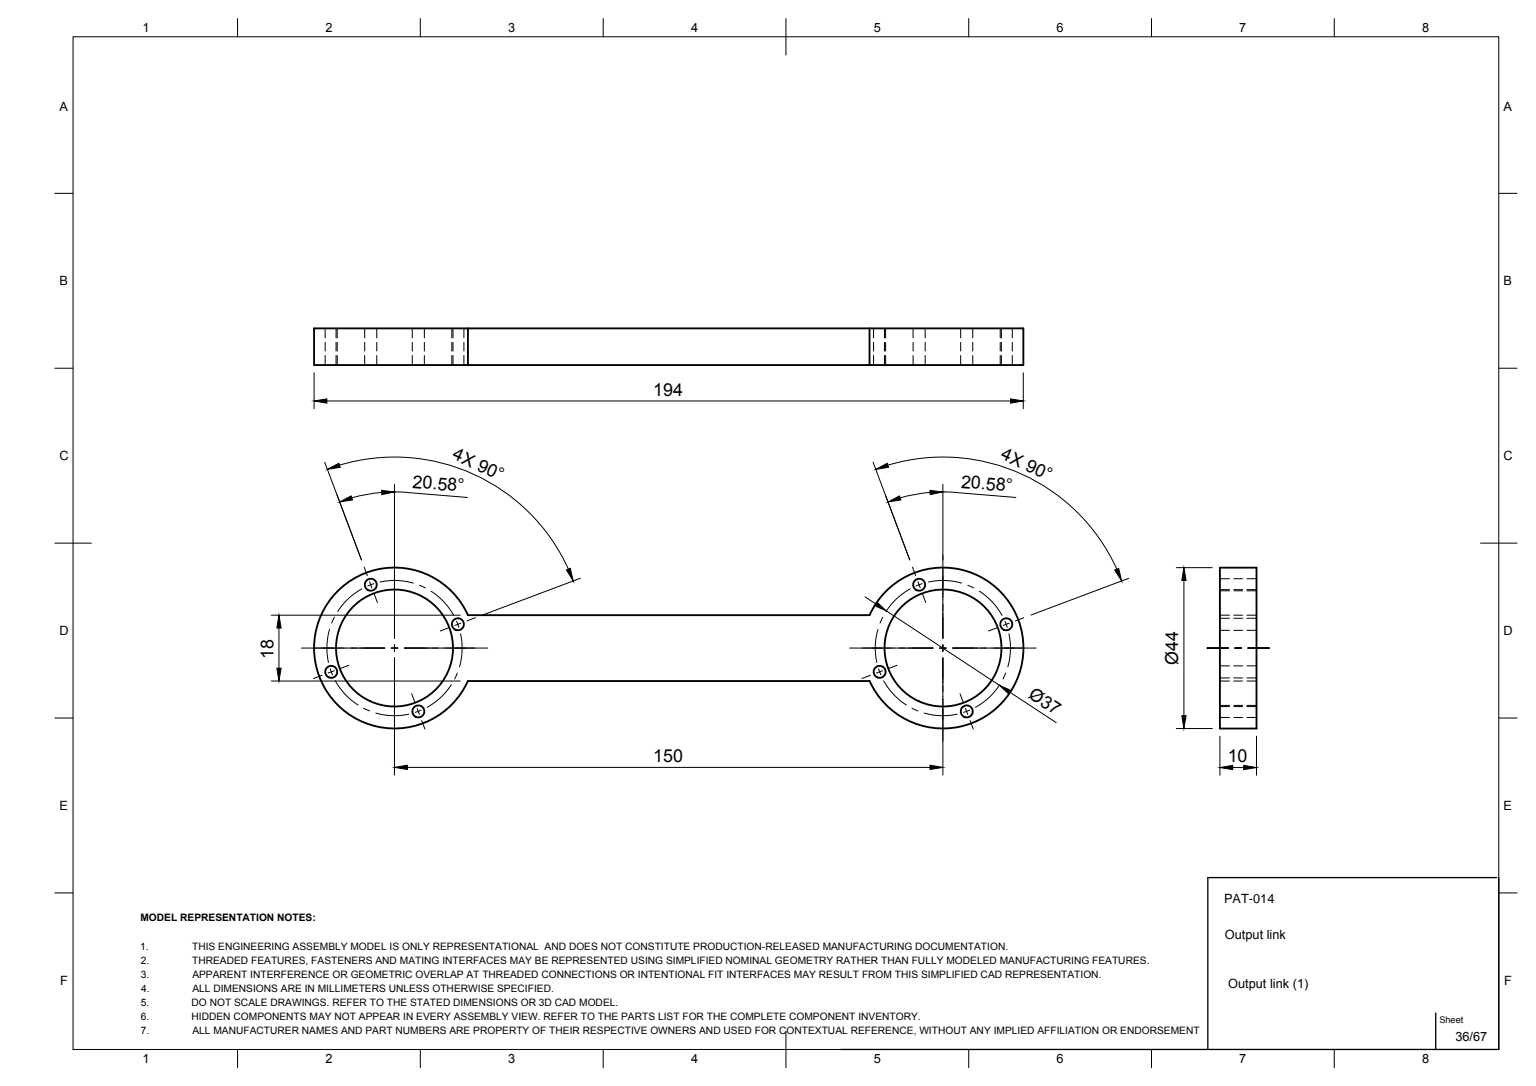
ISO-10303-21;
HEADER;
/* Generated by software containing ST-Developer
 * from STEP Tools, Inc. (www.steptools.com) 
 */

FILE_DESCRIPTION(
/* description */ ('Bin tilter linkage'),
/* implementation_level */ '2;1');

FILE_NAME(
/* name */ 'Output link (1).step',
/* time_stamp */ '2026-10-28T03:26:24-07:00',
/* author */ (''),
/* organization */ (''),
/* preprocessor_version */ 'ST-DEVELOPER v20.2',
/* originating_system */ 'Autodesk Translation Framework v15.17.0.0',
/* authorisation */ '');

FILE_SCHEMA (('AUTOMOTIVE_DESIGN { 1 0 10303 214 3 1 1 }'));
ENDSEC;

DATA;
#10=MECHANICAL_DESIGN_GEOMETRIC_PRESENTATION_REPRESENTATION('',(#913),#23728);
#701=SHAPE_REPRESENTATION_RELATIONSHIP('SRR','None',#24167,#807);
#807=ADVANCED_BREP_SHAPE_REPRESENTATION('',(#1026),#23667);
#913=STYLED_ITEM('',(#24779),#1026);
#1026=MANIFOLD_SOLID_BREP('Body1',#12444);
#1310=FACE_BOUND('',#3275,.T.);
#1311=FACE_BOUND('',#3276,.T.);
#1312=FACE_BOUND('',#3277,.T.);
#1313=FACE_BOUND('',#3278,.T.);
#1314=FACE_BOUND('',#3279,.T.);
#1315=FACE_BOUND('',#3280,.T.);
#1316=FACE_BOUND('',#3281,.T.);
#1317=FACE_BOUND('',#3282,.T.);
#1318=FACE_BOUND('',#3283,.T.);
#1319=FACE_BOUND('',#3284,.T.);
#1320=FACE_BOUND('',#3293,.T.);
#1321=FACE_BOUND('',#3294,.T.);
#1322=FACE_BOUND('',#3295,.T.);
#1323=FACE_BOUND('',#3296,.T.);
#1324=FACE_BOUND('',#3297,.T.);
#1325=FACE_BOUND('',#3298,.T.);
#1326=FACE_BOUND('',#3299,.T.);
#1327=FACE_BOUND('',#3300,.T.);
#1328=FACE_BOUND('',#3301,.T.);
#1329=FACE_BOUND('',#3302,.T.);
#1677=PLANE('',#14507);
#1678=PLANE('',#14508);
#1679=PLANE('',#14527);
#1680=PLANE('',#14528);
#2267=FACE_OUTER_BOUND('',#3267,.T.);
#2268=FACE_OUTER_BOUND('',#3268,.T.);
#2269=FACE_OUTER_BOUND('',#3269,.T.);
#2270=FACE_OUTER_BOUND('',#3270,.T.);
#2271=FACE_OUTER_BOUND('',#3271,.T.);
#2272=FACE_OUTER_BOUND('',#3272,.T.);
#2273=FACE_OUTER_BOUND('',#3273,.T.);
#2274=FACE_OUTER_BOUND('',#3274,.T.);
#2275=FACE_OUTER_BOUND('',#3285,.T.);
#2276=FACE_OUTER_BOUND('',#3286,.T.);
#2277=FACE_OUTER_BOUND('',#3287,.T.);
#2278=FACE_OUTER_BOUND('',#3288,.T.);
#2279=FACE_OUTER_BOUND('',#3289,.T.);
#2280=FACE_OUTER_BOUND('',#3290,.T.);
#2281=FACE_OUTER_BOUND('',#3291,.T.);
#2282=FACE_OUTER_BOUND('',#3292,.T.);
#3267=EDGE_LOOP('',(#9793,#9794,#9795,#9796));
#3268=EDGE_LOOP('',(#9797,#9798,#9799,#9800));
#3269=EDGE_LOOP('',(#9801,#9802,#9803,#9804));
#3270=EDGE_LOOP('',(#9805,#9806,#9807,#9808));
#3271=EDGE_LOOP('',(#9809,#9810,#9811,#9812));
#3272=EDGE_LOOP('',(#9813,#9814,#9815,#9816));
#3273=EDGE_LOOP('',(#9817,#9818,#9819,#9820));
#3274=EDGE_LOOP('',(#9821,#9822,#9823,#9824));
#3275=EDGE_LOOP('',(#9825));
#3276=EDGE_LOOP('',(#9826));
#3277=EDGE_LOOP('',(#9827));
#3278=EDGE_LOOP('',(#9828));
#3279=EDGE_LOOP('',(#9829));
#3280=EDGE_LOOP('',(#9830));
#3281=EDGE_LOOP('',(#9831));
#3282=EDGE_LOOP('',(#9832));
#3283=EDGE_LOOP('',(#9833));
#3284=EDGE_LOOP('',(#9834));
#3285=EDGE_LOOP('',(#9835,#9836,#9837,#9838));
#3286=EDGE_LOOP('',(#9839,#9840,#9841,#9842));
#3287=EDGE_LOOP('',(#9843,#9844,#9845,#9846));
#3288=EDGE_LOOP('',(#9847,#9848,#9849,#9850));
#3289=EDGE_LOOP('',(#9851,#9852,#9853,#9854));
#3290=EDGE_LOOP('',(#9855,#9856,#9857,#9858));
#3291=EDGE_LOOP('',(#9859,#9860,#9861,#9862));
#3292=EDGE_LOOP('',(#9863,#9864,#9865,#9866));
#3293=EDGE_LOOP('',(#9867));
#3294=EDGE_LOOP('',(#9868));
#3295=EDGE_LOOP('',(#9869));
#3296=EDGE_LOOP('',(#9870));
#3297=EDGE_LOOP('',(#9871));
#3298=EDGE_LOOP('',(#9872));
#3299=EDGE_LOOP('',(#9873));
#3300=EDGE_LOOP('',(#9874));
#3301=EDGE_LOOP('',(#9875));
#3302=EDGE_LOOP('',(#9876));
#4179=LINE('',#21364,#4854);
#4180=LINE('',#21370,#4855);
#4181=LINE('',#21376,#4856);
#4182=LINE('',#21382,#4857);
#4183=LINE('',#21388,#4858);
#4184=LINE('',#21393,#4859);
#4185=LINE('',#21397,#4860);
#4186=LINE('',#21401,#4861);
#4187=LINE('',#21403,#4862);
#4188=LINE('',#21404,#4863);
#4189=LINE('',#21407,#4864);
#4190=LINE('',#21422,#4865);
#4191=LINE('',#21426,#4866);
#4192=LINE('',#21430,#4867);
#4193=LINE('',#21434,#4868);
#4194=LINE('',#21438,#4869);
#4195=LINE('',#21441,#4870);
#4196=LINE('',#21444,#4871);
#4854=VECTOR('',#17434,0.164999999999999);
#4855=VECTOR('',#17441,0.164999999999999);
#4856=VECTOR('',#17448,0.164999999999999);
#4857=VECTOR('',#17455,0.164999999999999);
#4858=VECTOR('',#17462,1.6);
#4859=VECTOR('',#17467,1.);
#4860=VECTOR('',#17470,1.);
#4861=VECTOR('',#17475,1.);
#4862=VECTOR('',#17476,1.);
#4863=VECTOR('',#17477,1.);
#4864=VECTOR('',#17480,1.);
#4865=VECTOR('',#17497,0.164999999999999);
#4866=VECTOR('',#17502,0.164999999999999);
#4867=VECTOR('',#17507,0.164999999999999);
#4868=VECTOR('',#17512,0.164999999999999);
#4869=VECTOR('',#17517,1.6);
#4870=VECTOR('',#17520,1.);
#4871=VECTOR('',#17525,1.);
#5579=CIRCLE('',#14490,0.164999999999999);
#5580=CIRCLE('',#14491,0.164999999999999);
#5581=CIRCLE('',#14493,0.164999999999999);
#5582=CIRCLE('',#14494,0.164999999999999);
#5583=CIRCLE('',#14496,0.164999999999999);
#5584=CIRCLE('',#14497,0.164999999999999);
#5585=CIRCLE('',#14499,0.164999999999999);
#5586=CIRCLE('',#14500,0.164999999999999);
#5587=CIRCLE('',#14502,1.6);
#5588=CIRCLE('',#14503,1.6);
#5589=CIRCLE('',#14505,2.2);
#5590=CIRCLE('',#14506,2.2);
#5591=CIRCLE('',#14509,2.2);
#5592=CIRCLE('',#14510,1.6);
#5593=CIRCLE('',#14511,0.164999999999999);
#5594=CIRCLE('',#14512,0.164999999999999);
#5595=CIRCLE('',#14513,0.164999999999999);
#5596=CIRCLE('',#14514,0.164999999999999);
#5597=CIRCLE('',#14516,0.164999999999999);
#5598=CIRCLE('',#14518,0.164999999999999);
#5599=CIRCLE('',#14520,0.164999999999999);
#5600=CIRCLE('',#14522,0.164999999999999);
#5601=CIRCLE('',#14524,1.6);
#5602=CIRCLE('',#14526,2.2);
#6429=VERTEX_POINT('',#21361);
#6430=VERTEX_POINT('',#21363);
#6431=VERTEX_POINT('',#21367);
#6432=VERTEX_POINT('',#21369);
#6433=VERTEX_POINT('',#21373);
#6434=VERTEX_POINT('',#21375);
#6435=VERTEX_POINT('',#21379);
#6436=VERTEX_POINT('',#21381);
#6437=VERTEX_POINT('',#21385);
#6438=VERTEX_POINT('',#21387);
#6439=VERTEX_POINT('',#21391);
#6440=VERTEX_POINT('',#21392);
#6441=VERTEX_POINT('',#21394);
#6442=VERTEX_POINT('',#21396);
#6443=VERTEX_POINT('',#21400);
#6444=VERTEX_POINT('',#21402);
#6445=VERTEX_POINT('',#21406);
#6446=VERTEX_POINT('',#21409);
#6447=VERTEX_POINT('',#21411);
#6448=VERTEX_POINT('',#21413);
#6449=VERTEX_POINT('',#21415);
#6450=VERTEX_POINT('',#21417);
#6451=VERTEX_POINT('',#21420);
#6452=VERTEX_POINT('',#21424);
#6453=VERTEX_POINT('',#21428);
#6454=VERTEX_POINT('',#21432);
#6455=VERTEX_POINT('',#21436);
#6456=VERTEX_POINT('',#21440);
#7636=EDGE_CURVE('',#6429,#6429,#5579,.T.);
#7637=EDGE_CURVE('',#6429,#6430,#4179,.T.);
#7638=EDGE_CURVE('',#6430,#6430,#5580,.T.);
#7639=EDGE_CURVE('',#6431,#6431,#5581,.T.);
#7640=EDGE_CURVE('',#6431,#6432,#4180,.T.);
#7641=EDGE_CURVE('',#6432,#6432,#5582,.T.);
#7642=EDGE_CURVE('',#6433,#6433,#5583,.T.);
#7643=EDGE_CURVE('',#6433,#6434,#4181,.T.);
#7644=EDGE_CURVE('',#6434,#6434,#5584,.T.);
#7645=EDGE_CURVE('',#6435,#6435,#5585,.T.);
#7646=EDGE_CURVE('',#6435,#6436,#4182,.T.);
#7647=EDGE_CURVE('',#6436,#6436,#5586,.T.);
#7648=EDGE_CURVE('',#6437,#6437,#5587,.T.);
#7649=EDGE_CURVE('',#6437,#6438,#4183,.T.);
#7650=EDGE_CURVE('',#6438,#6438,#5588,.T.);
#7651=EDGE_CURVE('',#6439,#6440,#4184,.T.);
#7652=EDGE_CURVE('',#6439,#6441,#5589,.T.);
#7653=EDGE_CURVE('',#6442,#6441,#4185,.T.);
#7654=EDGE_CURVE('',#6440,#6442,#5590,.T.);
#7655=EDGE_CURVE('',#6443,#6440,#4186,.T.);
#7656=EDGE_CURVE('',#6443,#6444,#4187,.T.);
#7657=EDGE_CURVE('',#6444,#6439,#4188,.T.);
#7658=EDGE_CURVE('',#6442,#6445,#4189,.T.);
#7659=EDGE_CURVE('',#6445,#6443,#5591,.T.);
#7660=EDGE_CURVE('',#6446,#6446,#5592,.T.);
#7661=EDGE_CURVE('',#6447,#6447,#5593,.T.);
#7662=EDGE_CURVE('',#6448,#6448,#5594,.T.);
#7663=EDGE_CURVE('',#6449,#6449,#5595,.T.);
#7664=EDGE_CURVE('',#6450,#6450,#5596,.T.);
#7665=EDGE_CURVE('',#6451,#6451,#5597,.T.);
#7666=EDGE_CURVE('',#6451,#6450,#4190,.T.);
#7667=EDGE_CURVE('',#6452,#6452,#5598,.T.);
#7668=EDGE_CURVE('',#6452,#6449,#4191,.T.);
#7669=EDGE_CURVE('',#6453,#6453,#5599,.T.);
#7670=EDGE_CURVE('',#6453,#6448,#4192,.T.);
#7671=EDGE_CURVE('',#6454,#6454,#5600,.T.);
#7672=EDGE_CURVE('',#6454,#6447,#4193,.T.);
#7673=EDGE_CURVE('',#6455,#6455,#5601,.T.);
#7674=EDGE_CURVE('',#6455,#6446,#4194,.T.);
#7675=EDGE_CURVE('',#6456,#6445,#4195,.T.);
#7676=EDGE_CURVE('',#6456,#6444,#5602,.T.);
#7677=EDGE_CURVE('',#6441,#6456,#4196,.T.);
#9793=ORIENTED_EDGE('',*,*,#7636,.F.);
#9794=ORIENTED_EDGE('',*,*,#7637,.T.);
#9795=ORIENTED_EDGE('',*,*,#7638,.F.);
#9796=ORIENTED_EDGE('',*,*,#7637,.F.);
#9797=ORIENTED_EDGE('',*,*,#7639,.F.);
#9798=ORIENTED_EDGE('',*,*,#7640,.T.);
#9799=ORIENTED_EDGE('',*,*,#7641,.F.);
#9800=ORIENTED_EDGE('',*,*,#7640,.F.);
#9801=ORIENTED_EDGE('',*,*,#7642,.F.);
#9802=ORIENTED_EDGE('',*,*,#7643,.T.);
#9803=ORIENTED_EDGE('',*,*,#7644,.F.);
#9804=ORIENTED_EDGE('',*,*,#7643,.F.);
#9805=ORIENTED_EDGE('',*,*,#7645,.F.);
#9806=ORIENTED_EDGE('',*,*,#7646,.T.);
#9807=ORIENTED_EDGE('',*,*,#7647,.F.);
#9808=ORIENTED_EDGE('',*,*,#7646,.F.);
#9809=ORIENTED_EDGE('',*,*,#7648,.F.);
#9810=ORIENTED_EDGE('',*,*,#7649,.T.);
#9811=ORIENTED_EDGE('',*,*,#7650,.F.);
#9812=ORIENTED_EDGE('',*,*,#7649,.F.);
#9813=ORIENTED_EDGE('',*,*,#7651,.F.);
#9814=ORIENTED_EDGE('',*,*,#7652,.T.);
#9815=ORIENTED_EDGE('',*,*,#7653,.F.);
#9816=ORIENTED_EDGE('',*,*,#7654,.F.);
#9817=ORIENTED_EDGE('',*,*,#7651,.T.);
#9818=ORIENTED_EDGE('',*,*,#7655,.F.);
#9819=ORIENTED_EDGE('',*,*,#7656,.T.);
#9820=ORIENTED_EDGE('',*,*,#7657,.T.);
#9821=ORIENTED_EDGE('',*,*,#7654,.T.);
#9822=ORIENTED_EDGE('',*,*,#7658,.T.);
#9823=ORIENTED_EDGE('',*,*,#7659,.T.);
#9824=ORIENTED_EDGE('',*,*,#7655,.T.);
#9825=ORIENTED_EDGE('',*,*,#7660,.T.);
#9826=ORIENTED_EDGE('',*,*,#7661,.T.);
#9827=ORIENTED_EDGE('',*,*,#7662,.T.);
#9828=ORIENTED_EDGE('',*,*,#7663,.T.);
#9829=ORIENTED_EDGE('',*,*,#7664,.T.);
#9830=ORIENTED_EDGE('',*,*,#7650,.T.);
#9831=ORIENTED_EDGE('',*,*,#7647,.T.);
#9832=ORIENTED_EDGE('',*,*,#7644,.T.);
#9833=ORIENTED_EDGE('',*,*,#7641,.T.);
#9834=ORIENTED_EDGE('',*,*,#7638,.T.);
#9835=ORIENTED_EDGE('',*,*,#7665,.F.);
#9836=ORIENTED_EDGE('',*,*,#7666,.T.);
#9837=ORIENTED_EDGE('',*,*,#7664,.F.);
#9838=ORIENTED_EDGE('',*,*,#7666,.F.);
#9839=ORIENTED_EDGE('',*,*,#7667,.F.);
#9840=ORIENTED_EDGE('',*,*,#7668,.T.);
#9841=ORIENTED_EDGE('',*,*,#7663,.F.);
#9842=ORIENTED_EDGE('',*,*,#7668,.F.);
#9843=ORIENTED_EDGE('',*,*,#7669,.F.);
#9844=ORIENTED_EDGE('',*,*,#7670,.T.);
#9845=ORIENTED_EDGE('',*,*,#7662,.F.);
#9846=ORIENTED_EDGE('',*,*,#7670,.F.);
#9847=ORIENTED_EDGE('',*,*,#7671,.F.);
#9848=ORIENTED_EDGE('',*,*,#7672,.T.);
#9849=ORIENTED_EDGE('',*,*,#7661,.F.);
#9850=ORIENTED_EDGE('',*,*,#7672,.F.);
#9851=ORIENTED_EDGE('',*,*,#7673,.F.);
#9852=ORIENTED_EDGE('',*,*,#7674,.T.);
#9853=ORIENTED_EDGE('',*,*,#7660,.F.);
#9854=ORIENTED_EDGE('',*,*,#7674,.F.);
#9855=ORIENTED_EDGE('',*,*,#7675,.F.);
#9856=ORIENTED_EDGE('',*,*,#7676,.T.);
#9857=ORIENTED_EDGE('',*,*,#7656,.F.);
#9858=ORIENTED_EDGE('',*,*,#7659,.F.);
#9859=ORIENTED_EDGE('',*,*,#7653,.T.);
#9860=ORIENTED_EDGE('',*,*,#7677,.T.);
#9861=ORIENTED_EDGE('',*,*,#7675,.T.);
#9862=ORIENTED_EDGE('',*,*,#7658,.F.);
#9863=ORIENTED_EDGE('',*,*,#7657,.F.);
#9864=ORIENTED_EDGE('',*,*,#7676,.F.);
#9865=ORIENTED_EDGE('',*,*,#7677,.F.);
#9866=ORIENTED_EDGE('',*,*,#7652,.F.);
#9867=ORIENTED_EDGE('',*,*,#7665,.T.);
#9868=ORIENTED_EDGE('',*,*,#7667,.T.);
#9869=ORIENTED_EDGE('',*,*,#7669,.T.);
#9870=ORIENTED_EDGE('',*,*,#7671,.T.);
#9871=ORIENTED_EDGE('',*,*,#7673,.T.);
#9872=ORIENTED_EDGE('',*,*,#7648,.T.);
#9873=ORIENTED_EDGE('',*,*,#7645,.T.);
#9874=ORIENTED_EDGE('',*,*,#7642,.T.);
#9875=ORIENTED_EDGE('',*,*,#7639,.T.);
#9876=ORIENTED_EDGE('',*,*,#7636,.T.);
#11455=CYLINDRICAL_SURFACE('',#14489,0.164999999999999);
#11456=CYLINDRICAL_SURFACE('',#14492,0.164999999999999);
#11457=CYLINDRICAL_SURFACE('',#14495,0.164999999999999);
#11458=CYLINDRICAL_SURFACE('',#14498,0.164999999999999);
#11459=CYLINDRICAL_SURFACE('',#14501,1.6);
#11460=CYLINDRICAL_SURFACE('',#14504,2.2);
#11461=CYLINDRICAL_SURFACE('',#14515,0.164999999999999);
#11462=CYLINDRICAL_SURFACE('',#14517,0.164999999999999);
#11463=CYLINDRICAL_SURFACE('',#14519,0.164999999999999);
#11464=CYLINDRICAL_SURFACE('',#14521,0.164999999999999);
#11465=CYLINDRICAL_SURFACE('',#14523,1.6);
#11466=CYLINDRICAL_SURFACE('',#14525,2.2);
#11992=ADVANCED_FACE('',(#2267),#11455,.F.);
#11993=ADVANCED_FACE('',(#2268),#11456,.F.);
#11994=ADVANCED_FACE('',(#2269),#11457,.F.);
#11995=ADVANCED_FACE('',(#2270),#11458,.F.);
#11996=ADVANCED_FACE('',(#2271),#11459,.F.);
#11997=ADVANCED_FACE('',(#2272),#11460,.T.);
#11998=ADVANCED_FACE('',(#2273),#1677,.T.);
#11999=ADVANCED_FACE('',(#2274,#1310,#1311,#1312,#1313,#1314,#1315,#1316,
#1317,#1318,#1319),#1678,.T.);
#12000=ADVANCED_FACE('',(#2275),#11461,.F.);
#12001=ADVANCED_FACE('',(#2276),#11462,.F.);
#12002=ADVANCED_FACE('',(#2277),#11463,.F.);
#12003=ADVANCED_FACE('',(#2278),#11464,.F.);
#12004=ADVANCED_FACE('',(#2279),#11465,.F.);
#12005=ADVANCED_FACE('',(#2280),#11466,.T.);
#12006=ADVANCED_FACE('',(#2281),#1679,.T.);
#12007=ADVANCED_FACE('',(#2282,#1320,#1321,#1322,#1323,#1324,#1325,#1326,
#1327,#1328,#1329),#1680,.F.);
#12444=CLOSED_SHELL('',(#11992,#11993,#11994,#11995,#11996,#11997,#11998,
#11999,#12000,#12001,#12002,#12003,#12004,#12005,#12006,#12007));
#14488=AXIS2_PLACEMENT_3D('',#21359,#17428,#17429);
#14489=AXIS2_PLACEMENT_3D('',#21360,#17430,#17431);
#14490=AXIS2_PLACEMENT_3D('',#21362,#17432,#17433);
#14491=AXIS2_PLACEMENT_3D('',#21365,#17435,#17436);
#14492=AXIS2_PLACEMENT_3D('',#21366,#17437,#17438);
#14493=AXIS2_PLACEMENT_3D('',#21368,#17439,#17440);
#14494=AXIS2_PLACEMENT_3D('',#21371,#17442,#17443);
#14495=AXIS2_PLACEMENT_3D('',#21372,#17444,#17445);
#14496=AXIS2_PLACEMENT_3D('',#21374,#17446,#17447);
#14497=AXIS2_PLACEMENT_3D('',#21377,#17449,#17450);
#14498=AXIS2_PLACEMENT_3D('',#21378,#17451,#17452);
#14499=AXIS2_PLACEMENT_3D('',#21380,#17453,#17454);
#14500=AXIS2_PLACEMENT_3D('',#21383,#17456,#17457);
#14501=AXIS2_PLACEMENT_3D('',#21384,#17458,#17459);
#14502=AXIS2_PLACEMENT_3D('',#21386,#17460,#17461);
#14503=AXIS2_PLACEMENT_3D('',#21389,#17463,#17464);
#14504=AXIS2_PLACEMENT_3D('',#21390,#17465,#17466);
#14505=AXIS2_PLACEMENT_3D('',#21395,#17468,#17469);
#14506=AXIS2_PLACEMENT_3D('',#21398,#17471,#17472);
#14507=AXIS2_PLACEMENT_3D('',#21399,#17473,#17474);
#14508=AXIS2_PLACEMENT_3D('',#21405,#17478,#17479);
#14509=AXIS2_PLACEMENT_3D('',#21408,#17481,#17482);
#14510=AXIS2_PLACEMENT_3D('',#21410,#17483,#17484);
#14511=AXIS2_PLACEMENT_3D('',#21412,#17485,#17486);
#14512=AXIS2_PLACEMENT_3D('',#21414,#17487,#17488);
#14513=AXIS2_PLACEMENT_3D('',#21416,#17489,#17490);
#14514=AXIS2_PLACEMENT_3D('',#21418,#17491,#17492);
#14515=AXIS2_PLACEMENT_3D('',#21419,#17493,#17494);
#14516=AXIS2_PLACEMENT_3D('',#21421,#17495,#17496);
#14517=AXIS2_PLACEMENT_3D('',#21423,#17498,#17499);
#14518=AXIS2_PLACEMENT_3D('',#21425,#17500,#17501);
#14519=AXIS2_PLACEMENT_3D('',#21427,#17503,#17504);
#14520=AXIS2_PLACEMENT_3D('',#21429,#17505,#17506);
#14521=AXIS2_PLACEMENT_3D('',#21431,#17508,#17509);
#14522=AXIS2_PLACEMENT_3D('',#21433,#17510,#17511);
#14523=AXIS2_PLACEMENT_3D('',#21435,#17513,#17514);
#14524=AXIS2_PLACEMENT_3D('',#21437,#17515,#17516);
#14525=AXIS2_PLACEMENT_3D('',#21439,#17518,#17519);
#14526=AXIS2_PLACEMENT_3D('',#21442,#17521,#17522);
#14527=AXIS2_PLACEMENT_3D('',#21443,#17523,#17524);
#14528=AXIS2_PLACEMENT_3D('',#21445,#17526,#17527);
#17428=DIRECTION('axis',(0.,0.,1.));
#17429=DIRECTION('refdir',(1.,0.,0.));
#17430=DIRECTION('center_axis',(0.,1.,0.));
#17431=DIRECTION('ref_axis',(1.,0.,0.));
#17432=DIRECTION('center_axis',(0.,1.,0.));
#17433=DIRECTION('ref_axis',(1.,0.,0.));
#17434=DIRECTION('',(0.,1.,0.));
#17435=DIRECTION('center_axis',(0.,-1.,0.));
#17436=DIRECTION('ref_axis',(1.,0.,0.));
#17437=DIRECTION('center_axis',(0.,1.,0.));
#17438=DIRECTION('ref_axis',(1.,0.,0.));
#17439=DIRECTION('center_axis',(0.,1.,0.));
#17440=DIRECTION('ref_axis',(1.,0.,0.));
#17441=DIRECTION('',(0.,1.,0.));
#17442=DIRECTION('center_axis',(0.,-1.,0.));
#17443=DIRECTION('ref_axis',(1.,0.,0.));
#17444=DIRECTION('center_axis',(0.,1.,0.));
#17445=DIRECTION('ref_axis',(1.,0.,0.));
#17446=DIRECTION('center_axis',(0.,1.,0.));
#17447=DIRECTION('ref_axis',(1.,0.,0.));
#17448=DIRECTION('',(0.,1.,0.));
#17449=DIRECTION('center_axis',(0.,-1.,0.));
#17450=DIRECTION('ref_axis',(1.,0.,0.));
#17451=DIRECTION('center_axis',(0.,1.,0.));
#17452=DIRECTION('ref_axis',(1.,0.,0.));
#17453=DIRECTION('center_axis',(0.,1.,0.));
#17454=DIRECTION('ref_axis',(1.,0.,0.));
#17455=DIRECTION('',(0.,1.,0.));
#17456=DIRECTION('center_axis',(0.,-1.,0.));
#17457=DIRECTION('ref_axis',(1.,0.,0.));
#17458=DIRECTION('center_axis',(0.,1.,0.));
#17459=DIRECTION('ref_axis',(1.,0.,0.));
#17460=DIRECTION('center_axis',(0.,1.,0.));
#17461=DIRECTION('ref_axis',(1.,0.,0.));
#17462=DIRECTION('',(0.,1.,0.));
#17463=DIRECTION('center_axis',(0.,-1.,0.));
#17464=DIRECTION('ref_axis',(1.,0.,0.));
#17465=DIRECTION('center_axis',(0.,1.,0.));
#17466=DIRECTION('ref_axis',(0.413471898601476,0.,0.910516880165816));
#17467=DIRECTION('',(0.,1.,0.));
#17468=DIRECTION('center_axis',(0.,1.,0.));
#17469=DIRECTION('ref_axis',(1.,0.,0.));
#17470=DIRECTION('',(0.,-1.,0.));
#17471=DIRECTION('center_axis',(0.,1.,0.));
#17472=DIRECTION('ref_axis',(1.,0.,0.));
#17473=DIRECTION('center_axis',(-0.910516880165816,0.,0.413471898601475));
#17474=DIRECTION('ref_axis',(0.413471898601475,0.,0.910516880165816));
#17475=DIRECTION('',(0.413471898601475,0.,0.910516880165816));
#17476=DIRECTION('',(0.,-1.,0.));
#17477=DIRECTION('',(0.413471898601475,0.,0.910516880165816));
#17478=DIRECTION('center_axis',(0.,1.,0.));
#17479=DIRECTION('ref_axis',(0.,0.,1.));
#17480=DIRECTION('',(-0.413471898601475,0.,-0.910516880165816));
#17481=DIRECTION('center_axis',(0.,1.,0.));
#17482=DIRECTION('ref_axis',(1.,0.,0.));
#17483=DIRECTION('center_axis',(0.,-1.,0.));
#17484=DIRECTION('ref_axis',(1.,0.,0.));
#17485=DIRECTION('center_axis',(0.,-1.,0.));
#17486=DIRECTION('ref_axis',(1.,0.,0.));
#17487=DIRECTION('center_axis',(0.,-1.,0.));
#17488=DIRECTION('ref_axis',(1.,0.,0.));
#17489=DIRECTION('center_axis',(0.,-1.,0.));
#17490=DIRECTION('ref_axis',(1.,0.,0.));
#17491=DIRECTION('center_axis',(0.,-1.,0.));
#17492=DIRECTION('ref_axis',(1.,0.,0.));
#17493=DIRECTION('center_axis',(0.,1.,0.));
#17494=DIRECTION('ref_axis',(1.,0.,0.));
#17495=DIRECTION('center_axis',(0.,1.,0.));
#17496=DIRECTION('ref_axis',(1.,0.,0.));
#17497=DIRECTION('',(0.,1.,0.));
#17498=DIRECTION('center_axis',(0.,1.,0.));
#17499=DIRECTION('ref_axis',(1.,0.,0.));
#17500=DIRECTION('center_axis',(0.,1.,0.));
#17501=DIRECTION('ref_axis',(1.,0.,0.));
#17502=DIRECTION('',(0.,1.,0.));
#17503=DIRECTION('center_axis',(0.,1.,0.));
#17504=DIRECTION('ref_axis',(1.,0.,0.));
#17505=DIRECTION('center_axis',(0.,1.,0.));
#17506=DIRECTION('ref_axis',(1.,0.,0.));
#17507=DIRECTION('',(0.,1.,0.));
#17508=DIRECTION('center_axis',(0.,1.,0.));
#17509=DIRECTION('ref_axis',(1.,0.,0.));
#17510=DIRECTION('center_axis',(0.,1.,0.));
#17511=DIRECTION('ref_axis',(1.,0.,0.));
#17512=DIRECTION('',(0.,1.,0.));
#17513=DIRECTION('center_axis',(0.,1.,0.));
#17514=DIRECTION('ref_axis',(1.,0.,0.));
#17515=DIRECTION('center_axis',(0.,1.,0.));
#17516=DIRECTION('ref_axis',(1.,0.,0.));
#17517=DIRECTION('',(0.,1.,0.));
#17518=DIRECTION('center_axis',(0.,1.,0.));
#17519=DIRECTION('ref_axis',(-0.413471898601474,0.,-0.910516880165817));
#17520=DIRECTION('',(0.,1.,0.));
#17521=DIRECTION('center_axis',(0.,1.,0.));
#17522=DIRECTION('ref_axis',(1.,0.,0.));
#17523=DIRECTION('center_axis',(0.910516880165816,0.,-0.413471898601475));
#17524=DIRECTION('ref_axis',(-0.413471898601475,0.,-0.910516880165816));
#17525=DIRECTION('',(-0.413471898601475,0.,-0.910516880165816));
#17526=DIRECTION('center_axis',(0.,1.,0.));
#17527=DIRECTION('ref_axis',(1.,0.,0.));
#21359=CARTESIAN_POINT('',(0.,0.,0.));
#21360=CARTESIAN_POINT('Origin',(22.893930933827,-0.6,27.3496056572921));
#21361=CARTESIAN_POINT('',(22.728930933827,-0.5,27.3496056572921));
#21362=CARTESIAN_POINT('Origin',(22.893930933827,-0.5,27.3496056572921));
#21363=CARTESIAN_POINT('',(22.728930933827,0.5,27.3496056572921));
#21364=CARTESIAN_POINT('',(22.728930933827,-0.6,27.3496056572921));
#21365=CARTESIAN_POINT('Origin',(22.893930933827,0.5,27.3496056572921));
#21366=CARTESIAN_POINT('Origin',(22.893930933827,-0.6,29.9659007476824));
#21367=CARTESIAN_POINT('',(22.728930933827,-0.5,29.9659007476824));
#21368=CARTESIAN_POINT('Origin',(22.893930933827,-0.5,29.9659007476824));
#21369=CARTESIAN_POINT('',(22.728930933827,0.5,29.9659007476824));
#21370=CARTESIAN_POINT('',(22.728930933827,-0.6,29.9659007476824));
#21371=CARTESIAN_POINT('Origin',(22.893930933827,0.5,29.9659007476824));
#21372=CARTESIAN_POINT('Origin',(25.5102260242172,-0.6,29.9659007476824));
#21373=CARTESIAN_POINT('',(25.3452260242172,-0.5,29.9659007476824));
#21374=CARTESIAN_POINT('Origin',(25.5102260242172,-0.5,29.9659007476824));
#21375=CARTESIAN_POINT('',(25.3452260242172,0.5,29.9659007476824));
#21376=CARTESIAN_POINT('',(25.3452260242172,-0.6,29.9659007476824));
#21377=CARTESIAN_POINT('Origin',(25.5102260242172,0.5,29.9659007476824));
#21378=CARTESIAN_POINT('Origin',(25.5102260242172,-0.6,27.3496056572921));
#21379=CARTESIAN_POINT('',(25.3452260242172,-0.5,27.3496056572921));
#21380=CARTESIAN_POINT('Origin',(25.5102260242172,-0.5,27.3496056572921));
#21381=CARTESIAN_POINT('',(25.3452260242172,0.5,27.3496056572921));
#21382=CARTESIAN_POINT('',(25.3452260242172,-0.6,27.3496056572921));
#21383=CARTESIAN_POINT('Origin',(25.5102260242172,0.5,27.3496056572921));
#21384=CARTESIAN_POINT('Origin',(24.2020784790221,-0.6,28.6577532024872));
#21385=CARTESIAN_POINT('',(22.6020784790221,-0.5,28.6577532024872));
#21386=CARTESIAN_POINT('Origin',(24.2020784790221,-0.5,28.6577532024872));
#21387=CARTESIAN_POINT('',(22.6020784790221,0.5,28.6577532024872));
#21388=CARTESIAN_POINT('',(22.6020784790221,-0.6,28.6577532024872));
#21389=CARTESIAN_POINT('Origin',(24.2020784790221,0.5,28.6577532024872));
#21390=CARTESIAN_POINT('Origin',(24.2020784790221,-0.5,28.6577532024872));
#21391=CARTESIAN_POINT('',(22.5525742431765,-0.5,27.2020280306477));
#21392=CARTESIAN_POINT('',(22.5525742431765,0.5,27.2020280306477));
#21393=CARTESIAN_POINT('',(22.5525742431765,-0.5,27.2020280306477));
#21394=CARTESIAN_POINT('',(24.191504627475,-0.5,26.457778613165));
#21395=CARTESIAN_POINT('Origin',(24.2020784790221,-0.5,28.6577532024872));
#21396=CARTESIAN_POINT('',(24.191504627475,0.5,26.457778613165));
#21397=CARTESIAN_POINT('',(24.191504627475,-0.5,26.457778613165));
#21398=CARTESIAN_POINT('Origin',(24.2020784790221,0.5,28.6577532024872));
#21399=CARTESIAN_POINT('Origin',(17.1805348078508,-0.5,15.3721247087413));
#21400=CARTESIAN_POINT('',(18.0105738515472,0.5,17.1999745893222));
#21401=CARTESIAN_POINT('',(17.1805348078508,0.5,15.3721247087413));
#21402=CARTESIAN_POINT('',(18.0105738515472,-0.5,17.1999745893222));
#21403=CARTESIAN_POINT('',(18.0105738515472,-0.5,17.1999745893222));
#21404=CARTESIAN_POINT('',(17.1805348078508,-0.5,15.3721247087413));
#21405=CARTESIAN_POINT('Origin',(21.1010392395111,0.5,21.8288766012436));
#21406=CARTESIAN_POINT('',(19.6495042358456,0.5,16.4557251718396));
#21407=CARTESIAN_POINT('',(25.0215436711714,0.5,28.2856284937459));
#21408=CARTESIAN_POINT('Origin',(18.,0.5,15.));
#21409=CARTESIAN_POINT('',(16.4,0.5,15.));
#21410=CARTESIAN_POINT('Origin',(18.,0.5,15.));
#21411=CARTESIAN_POINT('',(19.1431475451951,0.5,13.6918524548049));
#21412=CARTESIAN_POINT('Origin',(19.3081475451951,0.5,13.6918524548049));
#21413=CARTESIAN_POINT('',(19.1431475451951,0.5,16.3081475451951));
#21414=CARTESIAN_POINT('Origin',(19.3081475451951,0.5,16.3081475451951));
#21415=CARTESIAN_POINT('',(16.5268524548049,0.5,16.3081475451951));
#21416=CARTESIAN_POINT('Origin',(16.6918524548049,0.5,16.3081475451951));
#21417=CARTESIAN_POINT('',(16.5268524548049,0.5,13.6918524548049));
#21418=CARTESIAN_POINT('Origin',(16.6918524548049,0.5,13.6918524548049));
#21419=CARTESIAN_POINT('Origin',(16.6918524548049,-0.6,13.6918524548049));
#21420=CARTESIAN_POINT('',(16.5268524548049,-0.5,13.6918524548049));
#21421=CARTESIAN_POINT('Origin',(16.6918524548049,-0.5,13.6918524548049));
#21422=CARTESIAN_POINT('',(16.5268524548049,-0.6,13.6918524548049));
#21423=CARTESIAN_POINT('Origin',(16.6918524548049,-0.6,16.3081475451951));
#21424=CARTESIAN_POINT('',(16.5268524548049,-0.5,16.3081475451951));
#21425=CARTESIAN_POINT('Origin',(16.6918524548049,-0.5,16.3081475451951));
#21426=CARTESIAN_POINT('',(16.5268524548049,-0.6,16.3081475451951));
#21427=CARTESIAN_POINT('Origin',(19.3081475451951,-0.6,16.3081475451951));
#21428=CARTESIAN_POINT('',(19.1431475451951,-0.5,16.3081475451951));
#21429=CARTESIAN_POINT('Origin',(19.3081475451951,-0.5,16.3081475451951));
#21430=CARTESIAN_POINT('',(19.1431475451951,-0.6,16.3081475451951));
#21431=CARTESIAN_POINT('Origin',(19.3081475451951,-0.6,13.6918524548049));
#21432=CARTESIAN_POINT('',(19.1431475451951,-0.5,13.6918524548049));
#21433=CARTESIAN_POINT('Origin',(19.3081475451951,-0.5,13.6918524548049));
#21434=CARTESIAN_POINT('',(19.1431475451951,-0.6,13.6918524548049));
#21435=CARTESIAN_POINT('Origin',(18.,-0.6,15.));
#21436=CARTESIAN_POINT('',(16.4,-0.5,15.));
#21437=CARTESIAN_POINT('Origin',(18.,-0.5,15.));
#21438=CARTESIAN_POINT('',(16.4,-0.6,15.));
#21439=CARTESIAN_POINT('Origin',(18.,-0.5,15.));
#21440=CARTESIAN_POINT('',(19.6495042358456,-0.5,16.4557251718396));
#21441=CARTESIAN_POINT('',(19.6495042358456,-0.5,16.4557251718396));
#21442=CARTESIAN_POINT('Origin',(18.,-0.5,15.));
#21443=CARTESIAN_POINT('Origin',(25.0215436711714,-0.5,28.2856284937459));
#21444=CARTESIAN_POINT('',(25.0215436711714,-0.5,28.2856284937459));
#21445=CARTESIAN_POINT('Origin',(21.1010392395111,-0.5,21.8288766012436));
#23550=UNCERTAINTY_MEASURE_WITH_UNIT(LENGTH_MEASURE(0.001),#23729,
'DISTANCE_ACCURACY_VALUE',
'Maximum model space distance between geometric entities at asserted c
onnectivities');
#23611=UNCERTAINTY_MEASURE_WITH_UNIT(LENGTH_MEASURE(0.001),#23729,
'DISTANCE_ACCURACY_VALUE',
'Maximum model space distance between geometric entities at asserted c
onnectivities');
#23667=(
GEOMETRIC_REPRESENTATION_CONTEXT(3)
GLOBAL_UNCERTAINTY_ASSIGNED_CONTEXT((#23550))
GLOBAL_UNIT_ASSIGNED_CONTEXT((#23729,#23731,#23732))
REPRESENTATION_CONTEXT('','3D')
);
#23728=(
GEOMETRIC_REPRESENTATION_CONTEXT(3)
GLOBAL_UNCERTAINTY_ASSIGNED_CONTEXT((#23611))
GLOBAL_UNIT_ASSIGNED_CONTEXT((#23729,#23731,#23732))
REPRESENTATION_CONTEXT('','3D')
);
#23729=(
LENGTH_UNIT()
NAMED_UNIT(*)
SI_UNIT(.CENTI.,.METRE.)
);
#23731=(
NAMED_UNIT(*)
PLANE_ANGLE_UNIT()
SI_UNIT($,.RADIAN.)
);
#23732=(
NAMED_UNIT(*)
SI_UNIT($,.STERADIAN.)
SOLID_ANGLE_UNIT()
);
#23788=SHAPE_DEFINITION_REPRESENTATION(#23904,#24167);
#23904=PRODUCT_DEFINITION_SHAPE('',$,#24284);
#24167=SHAPE_REPRESENTATION('',(#14488),#23667);
#24228=PRODUCT_DEFINITION_CONTEXT('part definition',#24578,'design');
#24284=PRODUCT_DEFINITION('Output link (1)','Output link (1)',#24400,#24228);
#24400=PRODUCT_DEFINITION_FORMATION('',$,#24635);
#24578=APPLICATION_CONTEXT(
'Core Data for Automotive Mechanical Design Process');
#24579=PRODUCT_CONTEXT('part definition',#24578,'mechanical');
#24635=PRODUCT('Output link (1)','Output link (1)','Output link (1)',(#24579));
#24773=COLOUR_RGB('Off White',0.89,0.88,0.83);
#24774=FILL_AREA_STYLE_COLOUR('',#24773);
#24775=FILL_AREA_STYLE('',(#24774));
#24776=SURFACE_STYLE_FILL_AREA(#24775);
#24777=SURFACE_SIDE_STYLE('',(#24776));
#24778=SURFACE_STYLE_USAGE(.BOTH.,#24777);
#24779=PRESENTATION_STYLE_ASSIGNMENT((#24778));
ENDSEC;
END-ISO-10303-21;
